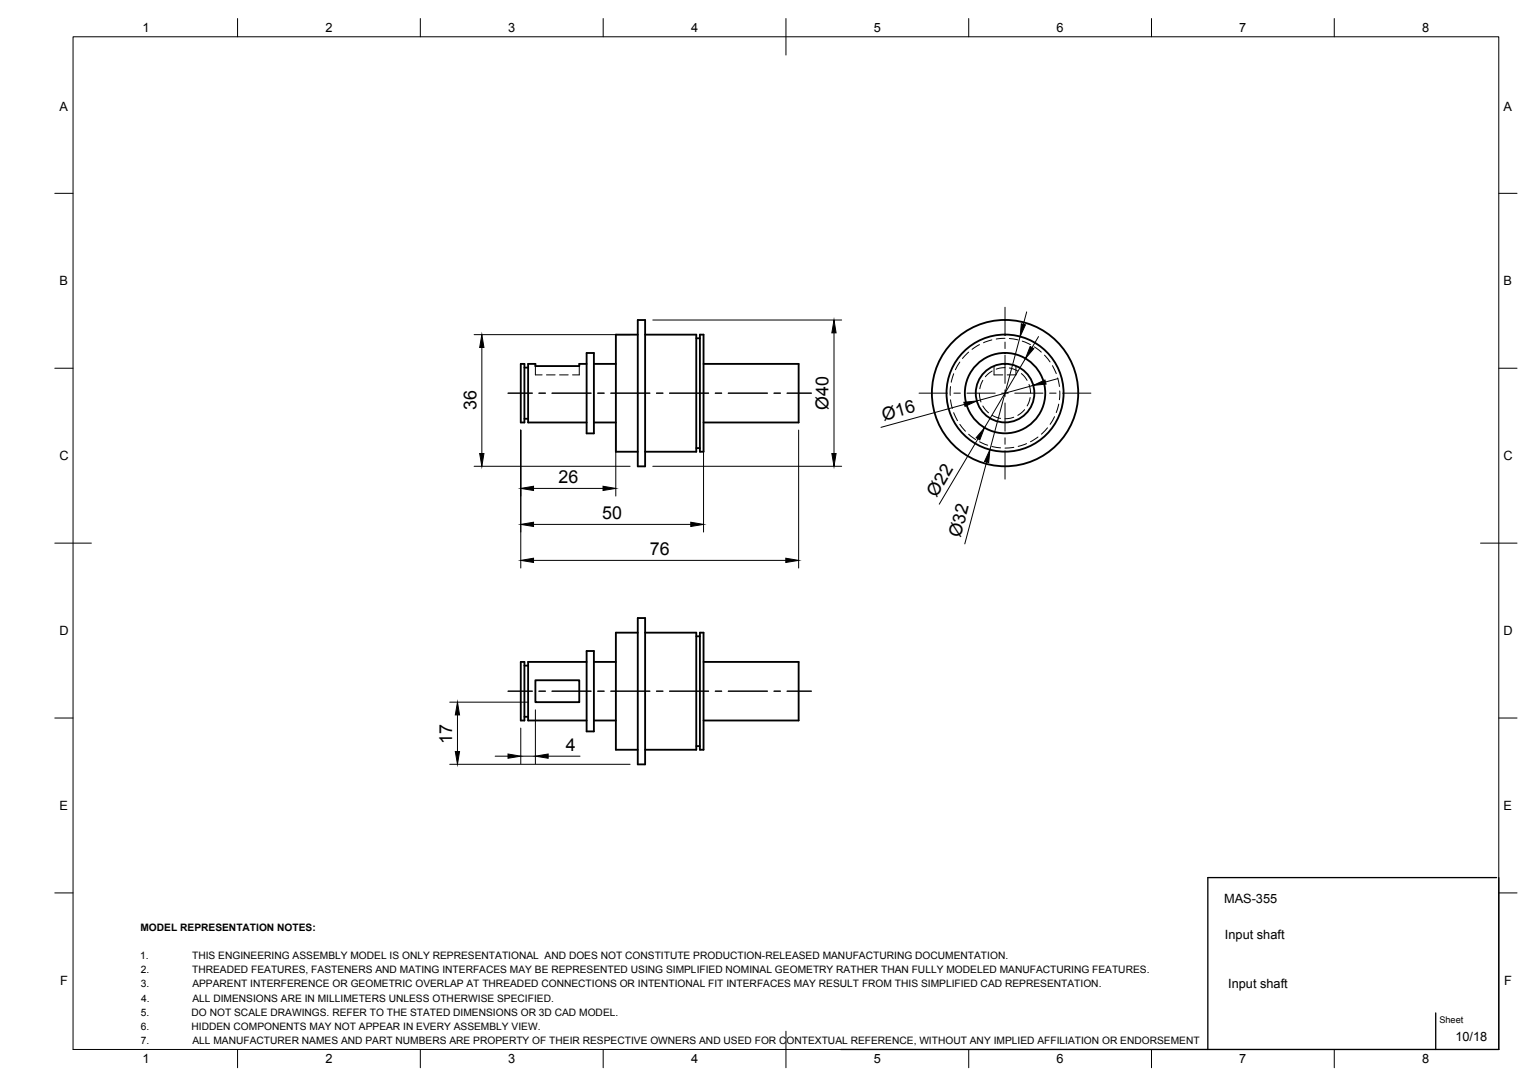
ISO-10303-21;
HEADER;
/* Generated by software containing ST-Developer
 * from STEP Tools, Inc. (www.steptools.com) 
 */

FILE_DESCRIPTION(
/* description */ ('Independent two-stage fixed-ring planetary gearbox,24/24/72 teeth,mod
ule2,20deg involutes,three planets per stage,4:1 x4:1=16:1. Native cut
-space/fillet/pattern tooth profiles derived from reusable gear blanks
; shared sun/planet/ring/carrier parts across both stages. Captured br
onze-journal input/carriers, headed retained planet pins, keyed inters
tage drive and modular keyed output interface. Native ideal gear links
; no torque, precision grade, production backlash/fits, lubrication, s
peed or life rating.'),
/* implementation_level */ '2;1');

FILE_NAME(
/* name */ 'Input shaft.step',
/* time_stamp */ '2026-11-08T19:10:00-08:00',
/* author */ (''),
/* organization */ (''),
/* preprocessor_version */ 'ST-DEVELOPER v20.2',
/* originating_system */ 'Autodesk Translation Framework v15.17.0.0',
/* authorisation */ '');

FILE_SCHEMA (('AUTOMOTIVE_DESIGN { 1 0 10303 214 3 1 1 }'));
ENDSEC;

DATA;
#10=MECHANICAL_DESIGN_GEOMETRIC_PRESENTATION_REPRESENTATION('',(#1166),#259224);
#1126=SHAPE_REPRESENTATION_RELATIONSHIP('SRR','None',#259373,#1146);
#1146=ADVANCED_BREP_SHAPE_REPRESENTATION('',(#1186),#259207);
#1166=STYLED_ITEM('',(#259482),#1186);
#1186=MANIFOLD_SOLID_BREP('Body1',#25153);
#1265=FACE_BOUND('',#3451,.T.);
#1266=FACE_BOUND('',#3453,.T.);
#1267=FACE_BOUND('',#3457,.T.);
#1268=FACE_BOUND('',#3459,.T.);
#1269=FACE_BOUND('',#3462,.T.);
#1270=FACE_BOUND('',#3464,.T.);
#1271=FACE_BOUND('',#3468,.T.);
#1272=FACE_BOUND('',#3470,.T.);
#1273=FACE_BOUND('',#3474,.T.);
#1274=FACE_BOUND('',#3480,.T.);
#1275=FACE_BOUND('',#3482,.T.);
#1509=PLANE('',#25812);
#1510=PLANE('',#25813);
#1511=PLANE('',#25815);
#1512=PLANE('',#25816);
#1513=PLANE('',#25817);
#1514=PLANE('',#25822);
#1515=PLANE('',#25824);
#1516=PLANE('',#25831);
#1517=PLANE('',#25833);
#1518=PLANE('',#25837);
#1519=PLANE('',#25840);
#1520=PLANE('',#25846);
#1521=PLANE('',#25849);
#1522=PLANE('',#25855);
#1523=PLANE('',#25859);
#1524=PLANE('',#25862);
#1525=PLANE('',#25863);
#2036=FACE_OUTER_BOUND('',#3444,.T.);
#2037=FACE_OUTER_BOUND('',#3445,.T.);
#2038=FACE_OUTER_BOUND('',#3446,.T.);
#2039=FACE_OUTER_BOUND('',#3447,.T.);
#2040=FACE_OUTER_BOUND('',#3448,.T.);
#2041=FACE_OUTER_BOUND('',#3449,.T.);
#2042=FACE_OUTER_BOUND('',#3450,.T.);
#2043=FACE_OUTER_BOUND('',#3452,.T.);
#2044=FACE_OUTER_BOUND('',#3454,.T.);
#2045=FACE_OUTER_BOUND('',#3455,.T.);
#2046=FACE_OUTER_BOUND('',#3456,.T.);
#2047=FACE_OUTER_BOUND('',#3458,.T.);
#2048=FACE_OUTER_BOUND('',#3460,.T.);
#2049=FACE_OUTER_BOUND('',#3461,.T.);
#2050=FACE_OUTER_BOUND('',#3463,.T.);
#2051=FACE_OUTER_BOUND('',#3465,.T.);
#2052=FACE_OUTER_BOUND('',#3466,.T.);
#2053=FACE_OUTER_BOUND('',#3467,.T.);
#2054=FACE_OUTER_BOUND('',#3469,.T.);
#2055=FACE_OUTER_BOUND('',#3471,.T.);
#2056=FACE_OUTER_BOUND('',#3472,.T.);
#2057=FACE_OUTER_BOUND('',#3473,.T.);
#2058=FACE_OUTER_BOUND('',#3475,.T.);
#2059=FACE_OUTER_BOUND('',#3476,.T.);
#2060=FACE_OUTER_BOUND('',#3477,.T.);
#2061=FACE_OUTER_BOUND('',#3478,.T.);
#2062=FACE_OUTER_BOUND('',#3479,.T.);
#2063=FACE_OUTER_BOUND('',#3481,.T.);
#3444=EDGE_LOOP('',(#17412,#17413,#17414,#17415));
#3445=EDGE_LOOP('',(#17416,#17417,#17418,#17419));
#3446=EDGE_LOOP('',(#17420,#17421,#17422,#17423));
#3447=EDGE_LOOP('',(#17424,#17425,#17426,#17427));
#3448=EDGE_LOOP('',(#17428,#17429,#17430,#17431));
#3449=EDGE_LOOP('',(#17432,#17433,#17434,#17435));
#3450=EDGE_LOOP('',(#17436));
#3451=EDGE_LOOP('',(#17437));
#3452=EDGE_LOOP('',(#17438));
#3453=EDGE_LOOP('',(#17439));
#3454=EDGE_LOOP('',(#17440,#17441,#17442,#17443));
#3455=EDGE_LOOP('',(#17444,#17445,#17446,#17447));
#3456=EDGE_LOOP('',(#17448));
#3457=EDGE_LOOP('',(#17449));
#3458=EDGE_LOOP('',(#17450));
#3459=EDGE_LOOP('',(#17451));
#3460=EDGE_LOOP('',(#17452,#17453,#17454,#17455));
#3461=EDGE_LOOP('',(#17456));
#3462=EDGE_LOOP('',(#17457));
#3463=EDGE_LOOP('',(#17458));
#3464=EDGE_LOOP('',(#17459));
#3465=EDGE_LOOP('',(#17460,#17461,#17462,#17463));
#3466=EDGE_LOOP('',(#17464,#17465,#17466,#17467));
#3467=EDGE_LOOP('',(#17468));
#3468=EDGE_LOOP('',(#17469));
#3469=EDGE_LOOP('',(#17470));
#3470=EDGE_LOOP('',(#17471));
#3471=EDGE_LOOP('',(#17472,#17473,#17474,#17475));
#3472=EDGE_LOOP('',(#17476,#17477,#17478,#17479));
#3473=EDGE_LOOP('',(#17480,#17481,#17482,#17483));
#3474=EDGE_LOOP('',(#17484,#17485,#17486,#17487));
#3475=EDGE_LOOP('',(#17488));
#3476=EDGE_LOOP('',(#17489,#17490,#17491,#17492));
#3477=EDGE_LOOP('',(#17493));
#3478=EDGE_LOOP('',(#17494,#17495,#17496,#17497));
#3479=EDGE_LOOP('',(#17498));
#3480=EDGE_LOOP('',(#17499));
#3481=EDGE_LOOP('',(#17500));
#3482=EDGE_LOOP('',(#17501));
#4599=CIRCLE('',#25814,8.);
#4600=CIRCLE('',#25818,8.);
#4601=CIRCLE('',#25820,7.);
#4602=CIRCLE('',#25821,7.);
#4603=CIRCLE('',#25823,8.);
#4604=CIRCLE('',#25825,8.);
#4605=CIRCLE('',#25827,8.);
#4606=CIRCLE('',#25829,15.);
#4607=CIRCLE('',#25830,15.);
#4608=CIRCLE('',#25832,16.);
#4609=CIRCLE('',#25834,16.);
#4610=CIRCLE('',#25836,16.);
#4611=CIRCLE('',#25838,11.);
#4612=CIRCLE('',#25839,8.);
#4613=CIRCLE('',#25841,11.);
#4614=CIRCLE('',#25842,8.);
#4615=CIRCLE('',#25845,8.);
#4616=CIRCLE('',#25847,20.);
#4617=CIRCLE('',#25848,16.);
#4618=CIRCLE('',#25850,20.);
#4619=CIRCLE('',#25853,16.);
#4620=CIRCLE('',#25857,8.);
#4621=CIRCLE('',#25858,8.);
#4622=CIRCLE('',#25861,16.);
#6959=LINE('',#52295,#8144);
#6960=LINE('',#52297,#8145);
#6961=LINE('',#52299,#8146);
#6962=LINE('',#52300,#8147);
#6963=LINE('',#52305,#8148);
#6964=LINE('',#52306,#8149);
#6965=LINE('',#52309,#8150);
#6966=LINE('',#52311,#8151);
#6967=LINE('',#52312,#8152);
#6968=LINE('',#52314,#8153);
#6969=LINE('',#52321,#8154);
#6970=LINE('',#52332,#8155);
#6971=LINE('',#52337,#8156);
#6972=LINE('',#52348,#8157);
#6973=LINE('',#52360,#8158);
#6974=LINE('',#52363,#8159);
#6975=LINE('',#52374,#8160);
#6976=LINE('',#52377,#8161);
#6977=LINE('',#52380,#8162);
#6978=LINE('',#52386,#8163);
#6979=LINE('',#52392,#8164);
#8144=VECTOR('',#28470,10.);
#8145=VECTOR('',#28471,10.);
#8146=VECTOR('',#28472,10.);
#8147=VECTOR('',#28473,10.);
#8148=VECTOR('',#28478,10.);
#8149=VECTOR('',#28479,10.);
#8150=VECTOR('',#28482,10.);
#8151=VECTOR('',#28483,10.);
#8152=VECTOR('',#28484,10.);
#8153=VECTOR('',#28487,10.);
#8154=VECTOR('',#28496,7.);
#8155=VECTOR('',#28511,8.);
#8156=VECTOR('',#28516,15.);
#8157=VECTOR('',#28531,16.);
#8158=VECTOR('',#28546,11.);
#8159=VECTOR('',#28549,8.);
#8160=VECTOR('',#28564,20.);
#8161=VECTOR('',#28567,16.);
#8162=VECTOR('',#28572,8.);
#8163=VECTOR('',#28579,8.);
#8164=VECTOR('',#28588,16.);
#9707=VERTEX_POINT('',#52293);
#9708=VERTEX_POINT('',#52294);
#9709=VERTEX_POINT('',#52296);
#9710=VERTEX_POINT('',#52298);
#9711=VERTEX_POINT('',#52302);
#9712=VERTEX_POINT('',#52304);
#9713=VERTEX_POINT('',#52308);
#9714=VERTEX_POINT('',#52310);
#9715=VERTEX_POINT('',#52318);
#9716=VERTEX_POINT('',#52320);
#9717=VERTEX_POINT('',#52324);
#9718=VERTEX_POINT('',#52327);
#9719=VERTEX_POINT('',#52330);
#9720=VERTEX_POINT('',#52334);
#9721=VERTEX_POINT('',#52336);
#9722=VERTEX_POINT('',#52340);
#9723=VERTEX_POINT('',#52343);
#9724=VERTEX_POINT('',#52346);
#9725=VERTEX_POINT('',#52350);
#9726=VERTEX_POINT('',#52352);
#9727=VERTEX_POINT('',#52355);
#9728=VERTEX_POINT('',#52357);
#9729=VERTEX_POINT('',#52362);
#9730=VERTEX_POINT('',#52366);
#9731=VERTEX_POINT('',#52368);
#9732=VERTEX_POINT('',#52371);
#9733=VERTEX_POINT('',#52376);
#9734=VERTEX_POINT('',#52383);
#9735=VERTEX_POINT('',#52385);
#9736=VERTEX_POINT('',#52390);
#12591=EDGE_CURVE('',#9707,#9708,#6959,.T.);
#12592=EDGE_CURVE('',#9707,#9709,#6960,.T.);
#12593=EDGE_CURVE('',#9710,#9709,#6961,.T.);
#12594=EDGE_CURVE('',#9710,#9708,#6962,.T.);
#12595=EDGE_CURVE('',#9708,#9711,#4599,.T.);
#12596=EDGE_CURVE('',#9712,#9710,#6963,.T.);
#12597=EDGE_CURVE('',#9711,#9712,#6964,.T.);
#12598=EDGE_CURVE('',#9711,#9713,#6965,.T.);
#12599=EDGE_CURVE('',#9712,#9714,#6966,.T.);
#12600=EDGE_CURVE('',#9714,#9713,#6967,.T.);
#12601=EDGE_CURVE('',#9709,#9714,#6968,.T.);
#12602=EDGE_CURVE('',#9713,#9707,#4600,.T.);
#12603=EDGE_CURVE('',#9715,#9715,#4601,.T.);
#12604=EDGE_CURVE('',#9715,#9716,#6969,.T.);
#12605=EDGE_CURVE('',#9716,#9716,#4602,.T.);
#12606=EDGE_CURVE('',#9717,#9717,#4603,.T.);
#12607=EDGE_CURVE('',#9718,#9718,#4604,.T.);
#12608=EDGE_CURVE('',#9719,#9719,#4605,.T.);
#12609=EDGE_CURVE('',#9719,#9718,#6970,.T.);
#12610=EDGE_CURVE('',#9720,#9720,#4606,.T.);
#12611=EDGE_CURVE('',#9720,#9721,#6971,.T.);
#12612=EDGE_CURVE('',#9721,#9721,#4607,.T.);
#12613=EDGE_CURVE('',#9722,#9722,#4608,.T.);
#12614=EDGE_CURVE('',#9723,#9723,#4609,.T.);
#12615=EDGE_CURVE('',#9724,#9724,#4610,.T.);
#12616=EDGE_CURVE('',#9724,#9723,#6972,.T.);
#12617=EDGE_CURVE('',#9725,#9725,#4611,.T.);
#12618=EDGE_CURVE('',#9726,#9726,#4612,.T.);
#12619=EDGE_CURVE('',#9727,#9727,#4613,.T.);
#12620=EDGE_CURVE('',#9728,#9728,#4614,.T.);
#12621=EDGE_CURVE('',#9725,#9727,#6973,.T.);
#12622=EDGE_CURVE('',#9728,#9729,#6974,.T.);
#12623=EDGE_CURVE('',#9729,#9729,#4615,.T.);
#12624=EDGE_CURVE('',#9730,#9730,#4616,.T.);
#12625=EDGE_CURVE('',#9731,#9731,#4617,.T.);
#12626=EDGE_CURVE('',#9732,#9732,#4618,.T.);
#12627=EDGE_CURVE('',#9730,#9732,#6975,.T.);
#12628=EDGE_CURVE('',#9722,#9733,#6976,.T.);
#12629=EDGE_CURVE('',#9733,#9733,#4619,.T.);
#12630=EDGE_CURVE('',#9717,#9726,#6977,.T.);
#12631=EDGE_CURVE('',#9734,#9734,#4620,.T.);
#12632=EDGE_CURVE('',#9734,#9735,#6978,.T.);
#12633=EDGE_CURVE('',#9735,#9735,#4621,.T.);
#12634=EDGE_CURVE('',#9736,#9736,#4622,.T.);
#12635=EDGE_CURVE('',#9736,#9731,#6979,.T.);
#17412=ORIENTED_EDGE('',*,*,#12591,.F.);
#17413=ORIENTED_EDGE('',*,*,#12592,.T.);
#17414=ORIENTED_EDGE('',*,*,#12593,.F.);
#17415=ORIENTED_EDGE('',*,*,#12594,.T.);
#17416=ORIENTED_EDGE('',*,*,#12595,.F.);
#17417=ORIENTED_EDGE('',*,*,#12594,.F.);
#17418=ORIENTED_EDGE('',*,*,#12596,.F.);
#17419=ORIENTED_EDGE('',*,*,#12597,.F.);
#17420=ORIENTED_EDGE('',*,*,#12598,.F.);
#17421=ORIENTED_EDGE('',*,*,#12597,.T.);
#17422=ORIENTED_EDGE('',*,*,#12599,.T.);
#17423=ORIENTED_EDGE('',*,*,#12600,.T.);
#17424=ORIENTED_EDGE('',*,*,#12596,.T.);
#17425=ORIENTED_EDGE('',*,*,#12593,.T.);
#17426=ORIENTED_EDGE('',*,*,#12601,.T.);
#17427=ORIENTED_EDGE('',*,*,#12599,.F.);
#17428=ORIENTED_EDGE('',*,*,#12602,.F.);
#17429=ORIENTED_EDGE('',*,*,#12600,.F.);
#17430=ORIENTED_EDGE('',*,*,#12601,.F.);
#17431=ORIENTED_EDGE('',*,*,#12592,.F.);
#17432=ORIENTED_EDGE('',*,*,#12603,.T.);
#17433=ORIENTED_EDGE('',*,*,#12604,.T.);
#17434=ORIENTED_EDGE('',*,*,#12605,.F.);
#17435=ORIENTED_EDGE('',*,*,#12604,.F.);
#17436=ORIENTED_EDGE('',*,*,#12606,.F.);
#17437=ORIENTED_EDGE('',*,*,#12603,.F.);
#17438=ORIENTED_EDGE('',*,*,#12607,.F.);
#17439=ORIENTED_EDGE('',*,*,#12605,.T.);
#17440=ORIENTED_EDGE('',*,*,#12608,.F.);
#17441=ORIENTED_EDGE('',*,*,#12609,.T.);
#17442=ORIENTED_EDGE('',*,*,#12607,.T.);
#17443=ORIENTED_EDGE('',*,*,#12609,.F.);
#17444=ORIENTED_EDGE('',*,*,#12610,.T.);
#17445=ORIENTED_EDGE('',*,*,#12611,.T.);
#17446=ORIENTED_EDGE('',*,*,#12612,.F.);
#17447=ORIENTED_EDGE('',*,*,#12611,.F.);
#17448=ORIENTED_EDGE('',*,*,#12613,.F.);
#17449=ORIENTED_EDGE('',*,*,#12610,.F.);
#17450=ORIENTED_EDGE('',*,*,#12614,.F.);
#17451=ORIENTED_EDGE('',*,*,#12612,.T.);
#17452=ORIENTED_EDGE('',*,*,#12615,.T.);
#17453=ORIENTED_EDGE('',*,*,#12616,.T.);
#17454=ORIENTED_EDGE('',*,*,#12614,.T.);
#17455=ORIENTED_EDGE('',*,*,#12616,.F.);
#17456=ORIENTED_EDGE('',*,*,#12617,.T.);
#17457=ORIENTED_EDGE('',*,*,#12618,.F.);
#17458=ORIENTED_EDGE('',*,*,#12619,.F.);
#17459=ORIENTED_EDGE('',*,*,#12620,.F.);
#17460=ORIENTED_EDGE('',*,*,#12617,.F.);
#17461=ORIENTED_EDGE('',*,*,#12621,.T.);
#17462=ORIENTED_EDGE('',*,*,#12619,.T.);
#17463=ORIENTED_EDGE('',*,*,#12621,.F.);
#17464=ORIENTED_EDGE('',*,*,#12620,.T.);
#17465=ORIENTED_EDGE('',*,*,#12622,.T.);
#17466=ORIENTED_EDGE('',*,*,#12623,.F.);
#17467=ORIENTED_EDGE('',*,*,#12622,.F.);
#17468=ORIENTED_EDGE('',*,*,#12624,.T.);
#17469=ORIENTED_EDGE('',*,*,#12625,.F.);
#17470=ORIENTED_EDGE('',*,*,#12626,.F.);
#17471=ORIENTED_EDGE('',*,*,#12615,.F.);
#17472=ORIENTED_EDGE('',*,*,#12624,.F.);
#17473=ORIENTED_EDGE('',*,*,#12627,.T.);
#17474=ORIENTED_EDGE('',*,*,#12626,.T.);
#17475=ORIENTED_EDGE('',*,*,#12627,.F.);
#17476=ORIENTED_EDGE('',*,*,#12613,.T.);
#17477=ORIENTED_EDGE('',*,*,#12628,.T.);
#17478=ORIENTED_EDGE('',*,*,#12629,.T.);
#17479=ORIENTED_EDGE('',*,*,#12628,.F.);
#17480=ORIENTED_EDGE('',*,*,#12606,.T.);
#17481=ORIENTED_EDGE('',*,*,#12630,.T.);
#17482=ORIENTED_EDGE('',*,*,#12618,.T.);
#17483=ORIENTED_EDGE('',*,*,#12630,.F.);
#17484=ORIENTED_EDGE('',*,*,#12598,.T.);
#17485=ORIENTED_EDGE('',*,*,#12602,.T.);
#17486=ORIENTED_EDGE('',*,*,#12591,.T.);
#17487=ORIENTED_EDGE('',*,*,#12595,.T.);
#17488=ORIENTED_EDGE('',*,*,#12608,.T.);
#17489=ORIENTED_EDGE('',*,*,#12631,.F.);
#17490=ORIENTED_EDGE('',*,*,#12632,.T.);
#17491=ORIENTED_EDGE('',*,*,#12633,.T.);
#17492=ORIENTED_EDGE('',*,*,#12632,.F.);
#17493=ORIENTED_EDGE('',*,*,#12633,.F.);
#17494=ORIENTED_EDGE('',*,*,#12634,.F.);
#17495=ORIENTED_EDGE('',*,*,#12635,.T.);
#17496=ORIENTED_EDGE('',*,*,#12625,.T.);
#17497=ORIENTED_EDGE('',*,*,#12635,.F.);
#17498=ORIENTED_EDGE('',*,*,#12634,.T.);
#17499=ORIENTED_EDGE('',*,*,#12623,.T.);
#17500=ORIENTED_EDGE('',*,*,#12629,.F.);
#17501=ORIENTED_EDGE('',*,*,#12631,.T.);
#23371=CYLINDRICAL_SURFACE('',#25819,7.);
#23372=CYLINDRICAL_SURFACE('',#25826,8.);
#23373=CYLINDRICAL_SURFACE('',#25828,15.);
#23374=CYLINDRICAL_SURFACE('',#25835,16.);
#23375=CYLINDRICAL_SURFACE('',#25843,11.);
#23376=CYLINDRICAL_SURFACE('',#25844,8.);
#23377=CYLINDRICAL_SURFACE('',#25851,20.);
#23378=CYLINDRICAL_SURFACE('',#25852,16.);
#23379=CYLINDRICAL_SURFACE('',#25854,8.);
#23380=CYLINDRICAL_SURFACE('',#25856,8.);
#23381=CYLINDRICAL_SURFACE('',#25860,16.);
#24142=ADVANCED_FACE('',(#2036),#1509,.F.);
#24143=ADVANCED_FACE('',(#2037),#1510,.F.);
#24144=ADVANCED_FACE('',(#2038),#1511,.F.);
#24145=ADVANCED_FACE('',(#2039),#1512,.F.);
#24146=ADVANCED_FACE('',(#2040),#1513,.F.);
#24147=ADVANCED_FACE('',(#2041),#23371,.T.);
#24148=ADVANCED_FACE('',(#2042,#1265),#1514,.F.);
#24149=ADVANCED_FACE('',(#2043,#1266),#1515,.F.);
#24150=ADVANCED_FACE('',(#2044),#23372,.T.);
#24151=ADVANCED_FACE('',(#2045),#23373,.T.);
#24152=ADVANCED_FACE('',(#2046,#1267),#1516,.F.);
#24153=ADVANCED_FACE('',(#2047,#1268),#1517,.F.);
#24154=ADVANCED_FACE('',(#2048),#23374,.T.);
#24155=ADVANCED_FACE('',(#2049,#1269),#1518,.T.);
#24156=ADVANCED_FACE('',(#2050,#1270),#1519,.F.);
#24157=ADVANCED_FACE('',(#2051),#23375,.T.);
#24158=ADVANCED_FACE('',(#2052),#23376,.T.);
#24159=ADVANCED_FACE('',(#2053,#1271),#1520,.T.);
#24160=ADVANCED_FACE('',(#2054,#1272),#1521,.F.);
#24161=ADVANCED_FACE('',(#2055),#23377,.T.);
#24162=ADVANCED_FACE('',(#2056),#23378,.T.);
#24163=ADVANCED_FACE('',(#2057,#1273),#23379,.T.);
#24164=ADVANCED_FACE('',(#2058),#1522,.T.);
#24165=ADVANCED_FACE('',(#2059),#23380,.T.);
#24166=ADVANCED_FACE('',(#2060),#1523,.F.);
#24167=ADVANCED_FACE('',(#2061),#23381,.T.);
#24168=ADVANCED_FACE('',(#2062,#1274),#1524,.T.);
#24169=ADVANCED_FACE('',(#2063,#1275),#1525,.F.);
#25153=CLOSED_SHELL('',(#24142,#24143,#24144,#24145,#24146,#24147,#24148,
#24149,#24150,#24151,#24152,#24153,#24154,#24155,#24156,#24157,#24158,#24159,
#24160,#24161,#24162,#24163,#24164,#24165,#24166,#24167,#24168,#24169));
#25811=AXIS2_PLACEMENT_3D('',#52291,#28466,#28467);
#25812=AXIS2_PLACEMENT_3D('',#52292,#28468,#28469);
#25813=AXIS2_PLACEMENT_3D('',#52301,#28474,#28475);
#25814=AXIS2_PLACEMENT_3D('',#52303,#28476,#28477);
#25815=AXIS2_PLACEMENT_3D('',#52307,#28480,#28481);
#25816=AXIS2_PLACEMENT_3D('',#52313,#28485,#28486);
#25817=AXIS2_PLACEMENT_3D('',#52315,#28488,#28489);
#25818=AXIS2_PLACEMENT_3D('',#52316,#28490,#28491);
#25819=AXIS2_PLACEMENT_3D('',#52317,#28492,#28493);
#25820=AXIS2_PLACEMENT_3D('',#52319,#28494,#28495);
#25821=AXIS2_PLACEMENT_3D('',#52322,#28497,#28498);
#25822=AXIS2_PLACEMENT_3D('',#52323,#28499,#28500);
#25823=AXIS2_PLACEMENT_3D('',#52325,#28501,#28502);
#25824=AXIS2_PLACEMENT_3D('',#52326,#28503,#28504);
#25825=AXIS2_PLACEMENT_3D('',#52328,#28505,#28506);
#25826=AXIS2_PLACEMENT_3D('',#52329,#28507,#28508);
#25827=AXIS2_PLACEMENT_3D('',#52331,#28509,#28510);
#25828=AXIS2_PLACEMENT_3D('',#52333,#28512,#28513);
#25829=AXIS2_PLACEMENT_3D('',#52335,#28514,#28515);
#25830=AXIS2_PLACEMENT_3D('',#52338,#28517,#28518);
#25831=AXIS2_PLACEMENT_3D('',#52339,#28519,#28520);
#25832=AXIS2_PLACEMENT_3D('',#52341,#28521,#28522);
#25833=AXIS2_PLACEMENT_3D('',#52342,#28523,#28524);
#25834=AXIS2_PLACEMENT_3D('',#52344,#28525,#28526);
#25835=AXIS2_PLACEMENT_3D('',#52345,#28527,#28528);
#25836=AXIS2_PLACEMENT_3D('',#52347,#28529,#28530);
#25837=AXIS2_PLACEMENT_3D('',#52349,#28532,#28533);
#25838=AXIS2_PLACEMENT_3D('',#52351,#28534,#28535);
#25839=AXIS2_PLACEMENT_3D('',#52353,#28536,#28537);
#25840=AXIS2_PLACEMENT_3D('',#52354,#28538,#28539);
#25841=AXIS2_PLACEMENT_3D('',#52356,#28540,#28541);
#25842=AXIS2_PLACEMENT_3D('',#52358,#28542,#28543);
#25843=AXIS2_PLACEMENT_3D('',#52359,#28544,#28545);
#25844=AXIS2_PLACEMENT_3D('',#52361,#28547,#28548);
#25845=AXIS2_PLACEMENT_3D('',#52364,#28550,#28551);
#25846=AXIS2_PLACEMENT_3D('',#52365,#28552,#28553);
#25847=AXIS2_PLACEMENT_3D('',#52367,#28554,#28555);
#25848=AXIS2_PLACEMENT_3D('',#52369,#28556,#28557);
#25849=AXIS2_PLACEMENT_3D('',#52370,#28558,#28559);
#25850=AXIS2_PLACEMENT_3D('',#52372,#28560,#28561);
#25851=AXIS2_PLACEMENT_3D('',#52373,#28562,#28563);
#25852=AXIS2_PLACEMENT_3D('',#52375,#28565,#28566);
#25853=AXIS2_PLACEMENT_3D('',#52378,#28568,#28569);
#25854=AXIS2_PLACEMENT_3D('',#52379,#28570,#28571);
#25855=AXIS2_PLACEMENT_3D('',#52381,#28573,#28574);
#25856=AXIS2_PLACEMENT_3D('',#52382,#28575,#28576);
#25857=AXIS2_PLACEMENT_3D('',#52384,#28577,#28578);
#25858=AXIS2_PLACEMENT_3D('',#52387,#28580,#28581);
#25859=AXIS2_PLACEMENT_3D('',#52388,#28582,#28583);
#25860=AXIS2_PLACEMENT_3D('',#52389,#28584,#28585);
#25861=AXIS2_PLACEMENT_3D('',#52391,#28586,#28587);
#25862=AXIS2_PLACEMENT_3D('',#52393,#28589,#28590);
#25863=AXIS2_PLACEMENT_3D('',#52394,#28591,#28592);
#28466=DIRECTION('axis',(0.,0.,1.));
#28467=DIRECTION('refdir',(1.,0.,0.));
#28468=DIRECTION('center_axis',(0.,-1.,0.));
#28469=DIRECTION('ref_axis',(-1.,0.,0.));
#28470=DIRECTION('',(0.,0.,1.));
#28471=DIRECTION('',(-1.,0.,0.));
#28472=DIRECTION('',(0.,0.,-1.));
#28473=DIRECTION('',(1.,0.,0.));
#28474=DIRECTION('center_axis',(0.,0.,1.));
#28475=DIRECTION('ref_axis',(1.,0.,0.));
#28476=DIRECTION('center_axis',(0.,0.,1.));
#28477=DIRECTION('ref_axis',(1.,0.,0.));
#28478=DIRECTION('',(0.,-1.,0.));
#28479=DIRECTION('',(-1.,0.,0.));
#28480=DIRECTION('center_axis',(0.,1.,0.));
#28481=DIRECTION('ref_axis',(1.,0.,0.));
#28482=DIRECTION('',(0.,0.,-1.));
#28483=DIRECTION('',(0.,0.,-1.));
#28484=DIRECTION('',(1.,0.,0.));
#28485=DIRECTION('center_axis',(-1.,0.,0.));
#28486=DIRECTION('ref_axis',(0.,1.,0.));
#28487=DIRECTION('',(0.,1.,0.));
#28488=DIRECTION('center_axis',(0.,0.,-1.));
#28489=DIRECTION('ref_axis',(-1.,0.,0.));
#28490=DIRECTION('center_axis',(0.,0.,-1.));
#28491=DIRECTION('ref_axis',(1.,0.,0.));
#28492=DIRECTION('center_axis',(0.,0.,1.));
#28493=DIRECTION('ref_axis',(1.,0.,0.));
#28494=DIRECTION('center_axis',(0.,0.,1.));
#28495=DIRECTION('ref_axis',(1.,0.,0.));
#28496=DIRECTION('',(0.,0.,1.));
#28497=DIRECTION('center_axis',(0.,0.,1.));
#28498=DIRECTION('ref_axis',(1.,0.,0.));
#28499=DIRECTION('center_axis',(0.,0.,-1.));
#28500=DIRECTION('ref_axis',(-1.,0.,0.));
#28501=DIRECTION('center_axis',(0.,0.,-1.));
#28502=DIRECTION('ref_axis',(1.,0.,0.));
#28503=DIRECTION('center_axis',(0.,0.,1.));
#28504=DIRECTION('ref_axis',(1.,0.,0.));
#28505=DIRECTION('center_axis',(0.,0.,1.));
#28506=DIRECTION('ref_axis',(1.,0.,0.));
#28507=DIRECTION('center_axis',(0.,0.,1.));
#28508=DIRECTION('ref_axis',(1.,0.,0.));
#28509=DIRECTION('center_axis',(0.,0.,1.));
#28510=DIRECTION('ref_axis',(1.,0.,0.));
#28511=DIRECTION('',(0.,0.,-1.));
#28512=DIRECTION('center_axis',(0.,0.,1.));
#28513=DIRECTION('ref_axis',(1.,0.,0.));
#28514=DIRECTION('center_axis',(0.,0.,1.));
#28515=DIRECTION('ref_axis',(1.,0.,0.));
#28516=DIRECTION('',(0.,0.,1.));
#28517=DIRECTION('center_axis',(0.,0.,1.));
#28518=DIRECTION('ref_axis',(1.,0.,0.));
#28519=DIRECTION('center_axis',(0.,0.,-1.));
#28520=DIRECTION('ref_axis',(-1.,0.,0.));
#28521=DIRECTION('center_axis',(0.,0.,-1.));
#28522=DIRECTION('ref_axis',(1.,0.,0.));
#28523=DIRECTION('center_axis',(0.,0.,1.));
#28524=DIRECTION('ref_axis',(1.,0.,0.));
#28525=DIRECTION('center_axis',(0.,0.,1.));
#28526=DIRECTION('ref_axis',(1.,0.,0.));
#28527=DIRECTION('center_axis',(0.,0.,1.));
#28528=DIRECTION('ref_axis',(1.,0.,0.));
#28529=DIRECTION('center_axis',(0.,0.,-1.));
#28530=DIRECTION('ref_axis',(1.,0.,0.));
#28531=DIRECTION('',(0.,0.,-1.));
#28532=DIRECTION('center_axis',(0.,0.,1.));
#28533=DIRECTION('ref_axis',(1.,0.,0.));
#28534=DIRECTION('center_axis',(0.,0.,1.));
#28535=DIRECTION('ref_axis',(1.,0.,0.));
#28536=DIRECTION('center_axis',(0.,0.,1.));
#28537=DIRECTION('ref_axis',(1.,0.,0.));
#28538=DIRECTION('center_axis',(0.,0.,1.));
#28539=DIRECTION('ref_axis',(1.,0.,0.));
#28540=DIRECTION('center_axis',(0.,0.,1.));
#28541=DIRECTION('ref_axis',(1.,0.,0.));
#28542=DIRECTION('center_axis',(0.,0.,-1.));
#28543=DIRECTION('ref_axis',(1.,0.,0.));
#28544=DIRECTION('center_axis',(0.,0.,1.));
#28545=DIRECTION('ref_axis',(1.,0.,0.));
#28546=DIRECTION('',(0.,0.,-1.));
#28547=DIRECTION('center_axis',(0.,0.,1.));
#28548=DIRECTION('ref_axis',(1.,0.,0.));
#28549=DIRECTION('',(0.,0.,-1.));
#28550=DIRECTION('center_axis',(0.,0.,-1.));
#28551=DIRECTION('ref_axis',(1.,0.,0.));
#28552=DIRECTION('center_axis',(0.,0.,1.));
#28553=DIRECTION('ref_axis',(1.,0.,0.));
#28554=DIRECTION('center_axis',(0.,0.,1.));
#28555=DIRECTION('ref_axis',(1.,0.,0.));
#28556=DIRECTION('center_axis',(0.,0.,1.));
#28557=DIRECTION('ref_axis',(1.,0.,0.));
#28558=DIRECTION('center_axis',(0.,0.,1.));
#28559=DIRECTION('ref_axis',(1.,0.,0.));
#28560=DIRECTION('center_axis',(0.,0.,1.));
#28561=DIRECTION('ref_axis',(1.,0.,0.));
#28562=DIRECTION('center_axis',(0.,0.,1.));
#28563=DIRECTION('ref_axis',(1.,0.,0.));
#28564=DIRECTION('',(0.,0.,-1.));
#28565=DIRECTION('center_axis',(0.,0.,1.));
#28566=DIRECTION('ref_axis',(1.,0.,0.));
#28567=DIRECTION('',(0.,0.,-1.));
#28568=DIRECTION('center_axis',(0.,0.,1.));
#28569=DIRECTION('ref_axis',(1.,0.,0.));
#28570=DIRECTION('center_axis',(0.,0.,1.));
#28571=DIRECTION('ref_axis',(1.,0.,0.));
#28572=DIRECTION('',(0.,0.,-1.));
#28573=DIRECTION('center_axis',(0.,0.,1.));
#28574=DIRECTION('ref_axis',(1.,0.,0.));
#28575=DIRECTION('center_axis',(0.,0.,1.));
#28576=DIRECTION('ref_axis',(1.,0.,0.));
#28577=DIRECTION('center_axis',(0.,0.,1.));
#28578=DIRECTION('ref_axis',(1.,0.,0.));
#28579=DIRECTION('',(0.,0.,-1.));
#28580=DIRECTION('center_axis',(0.,0.,1.));
#28581=DIRECTION('ref_axis',(1.,0.,0.));
#28582=DIRECTION('center_axis',(0.,0.,1.));
#28583=DIRECTION('ref_axis',(1.,0.,0.));
#28584=DIRECTION('center_axis',(0.,0.,1.));
#28585=DIRECTION('ref_axis',(1.,0.,0.));
#28586=DIRECTION('center_axis',(0.,0.,1.));
#28587=DIRECTION('ref_axis',(1.,0.,0.));
#28588=DIRECTION('',(0.,0.,-1.));
#28589=DIRECTION('center_axis',(0.,0.,1.));
#28590=DIRECTION('ref_axis',(1.,0.,0.));
#28591=DIRECTION('center_axis',(0.,0.,1.));
#28592=DIRECTION('ref_axis',(1.,0.,0.));
#52291=CARTESIAN_POINT('',(0.,0.,0.));
#52292=CARTESIAN_POINT('Origin',(11.,-3.,42.));
#52293=CARTESIAN_POINT('',(7.41619848709566,-3.,30.));
#52294=CARTESIAN_POINT('',(7.41619848709566,-3.,42.));
#52295=CARTESIAN_POINT('',(7.41619848709566,-3.,20.));
#52296=CARTESIAN_POINT('',(5.,-3.,30.));
#52297=CARTESIAN_POINT('',(5.,-3.,30.));
#52298=CARTESIAN_POINT('',(5.,-3.,42.));
#52299=CARTESIAN_POINT('',(5.,-3.,42.));
#52300=CARTESIAN_POINT('',(5.,-3.,42.));
#52301=CARTESIAN_POINT('Origin',(8.,0.,42.));
#52302=CARTESIAN_POINT('',(7.41619848709566,3.,42.));
#52303=CARTESIAN_POINT('Origin',(0.,0.,42.));
#52304=CARTESIAN_POINT('',(5.,3.,42.));
#52305=CARTESIAN_POINT('',(5.,3.,42.));
#52306=CARTESIAN_POINT('',(11.,3.,42.));
#52307=CARTESIAN_POINT('Origin',(5.,3.,42.));
#52308=CARTESIAN_POINT('',(7.41619848709566,3.,30.));
#52309=CARTESIAN_POINT('',(7.41619848709566,3.,20.));
#52310=CARTESIAN_POINT('',(5.,3.,30.));
#52311=CARTESIAN_POINT('',(5.,3.,42.));
#52312=CARTESIAN_POINT('',(11.,3.,30.));
#52313=CARTESIAN_POINT('Origin',(5.,-3.,42.));
#52314=CARTESIAN_POINT('',(5.,3.,30.));
#52315=CARTESIAN_POINT('Origin',(8.,0.,30.));
#52316=CARTESIAN_POINT('Origin',(0.,0.,30.));
#52317=CARTESIAN_POINT('Origin',(0.,0.,44.5));
#52318=CARTESIAN_POINT('',(-7.,-8.57252759403147E-16,44.));
#52319=CARTESIAN_POINT('Origin',(0.,0.,44.));
#52320=CARTESIAN_POINT('',(-7.,-8.57252759403147E-16,45.));
#52321=CARTESIAN_POINT('',(-7.,-8.57252759403147E-16,44.5));
#52322=CARTESIAN_POINT('Origin',(0.,0.,45.));
#52323=CARTESIAN_POINT('Origin',(11.,0.,44.));
#52324=CARTESIAN_POINT('',(-8.,9.79717439317883E-16,44.));
#52325=CARTESIAN_POINT('Origin',(0.,0.,44.));
#52326=CARTESIAN_POINT('Origin',(7.,0.,45.));
#52327=CARTESIAN_POINT('',(-8.,-9.79717439317883E-16,45.));
#52328=CARTESIAN_POINT('Origin',(0.,0.,45.));
#52329=CARTESIAN_POINT('Origin',(0.,0.,20.));
#52330=CARTESIAN_POINT('',(-8.,-9.79717439317883E-16,46.));
#52331=CARTESIAN_POINT('Origin',(0.,0.,46.));
#52332=CARTESIAN_POINT('',(-8.,-9.79717439317883E-16,20.));
#52333=CARTESIAN_POINT('Origin',(0.,0.,-2.5));
#52334=CARTESIAN_POINT('',(-15.,-1.83697019872103E-15,-3.));
#52335=CARTESIAN_POINT('Origin',(0.,0.,-3.));
#52336=CARTESIAN_POINT('',(-15.,-1.83697019872103E-15,-2.));
#52337=CARTESIAN_POINT('',(-15.,-1.83697019872103E-15,-2.5));
#52338=CARTESIAN_POINT('Origin',(0.,0.,-2.));
#52339=CARTESIAN_POINT('Origin',(19.,0.,-3.));
#52340=CARTESIAN_POINT('',(-16.,1.95943487863577E-15,-3.));
#52341=CARTESIAN_POINT('Origin',(0.,0.,-3.));
#52342=CARTESIAN_POINT('Origin',(15.,0.,-2.));
#52343=CARTESIAN_POINT('',(-16.,-1.95943487863577E-15,-2.));
#52344=CARTESIAN_POINT('Origin',(0.,0.,-2.));
#52345=CARTESIAN_POINT('Origin',(0.,0.,-4.));
#52346=CARTESIAN_POINT('',(-16.,1.95943487863577E-15,12.));
#52347=CARTESIAN_POINT('Origin',(0.,0.,12.));
#52348=CARTESIAN_POINT('',(-16.,-1.95943487863577E-15,-4.));
#52349=CARTESIAN_POINT('Origin',(0.,0.,28.));
#52350=CARTESIAN_POINT('',(-11.,-1.34711147906209E-15,28.));
#52351=CARTESIAN_POINT('Origin',(0.,0.,28.));
#52352=CARTESIAN_POINT('',(-8.,-9.79717439317883E-16,28.));
#52353=CARTESIAN_POINT('Origin',(0.,0.,28.));
#52354=CARTESIAN_POINT('Origin',(0.,0.,26.));
#52355=CARTESIAN_POINT('',(-11.,-1.34711147906209E-15,26.));
#52356=CARTESIAN_POINT('Origin',(0.,0.,26.));
#52357=CARTESIAN_POINT('',(-8.,9.79717439317883E-16,26.));
#52358=CARTESIAN_POINT('Origin',(0.,0.,26.));
#52359=CARTESIAN_POINT('Origin',(0.,0.,26.));
#52360=CARTESIAN_POINT('',(-11.,-1.34711147906209E-15,26.));
#52361=CARTESIAN_POINT('Origin',(0.,0.,20.));
#52362=CARTESIAN_POINT('',(-8.,-9.79717439317883E-16,20.));
#52363=CARTESIAN_POINT('',(-8.,-9.79717439317883E-16,20.));
#52364=CARTESIAN_POINT('Origin',(0.,0.,20.));
#52365=CARTESIAN_POINT('Origin',(0.,0.,14.));
#52366=CARTESIAN_POINT('',(-20.,-2.44929359829471E-15,14.));
#52367=CARTESIAN_POINT('Origin',(0.,0.,14.));
#52368=CARTESIAN_POINT('',(-16.,-1.95943487863577E-15,14.));
#52369=CARTESIAN_POINT('Origin',(0.,0.,14.));
#52370=CARTESIAN_POINT('Origin',(0.,0.,12.));
#52371=CARTESIAN_POINT('',(-20.,-2.44929359829471E-15,12.));
#52372=CARTESIAN_POINT('Origin',(0.,0.,12.));
#52373=CARTESIAN_POINT('Origin',(0.,0.,12.));
#52374=CARTESIAN_POINT('',(-20.,-2.44929359829471E-15,12.));
#52375=CARTESIAN_POINT('Origin',(0.,0.,-4.));
#52376=CARTESIAN_POINT('',(-16.,-1.95943487863577E-15,-4.));
#52377=CARTESIAN_POINT('',(-16.,-1.95943487863577E-15,-4.));
#52378=CARTESIAN_POINT('Origin',(0.,0.,-4.));
#52379=CARTESIAN_POINT('Origin',(0.,0.,20.));
#52380=CARTESIAN_POINT('',(-8.,-9.79717439317883E-16,20.));
#52381=CARTESIAN_POINT('Origin',(0.,0.,46.));
#52382=CARTESIAN_POINT('Origin',(0.,0.,-20.));
#52383=CARTESIAN_POINT('',(-8.,-9.79717439317883E-16,-4.));
#52384=CARTESIAN_POINT('Origin',(0.,0.,-4.));
#52385=CARTESIAN_POINT('',(-8.,-9.79717439317883E-16,-30.));
#52386=CARTESIAN_POINT('',(-8.,-9.79717439317883E-16,-20.));
#52387=CARTESIAN_POINT('Origin',(0.,0.,-30.));
#52388=CARTESIAN_POINT('Origin',(0.,0.,-30.));
#52389=CARTESIAN_POINT('Origin',(0.,0.,-4.));
#52390=CARTESIAN_POINT('',(-16.,-1.95943487863577E-15,20.));
#52391=CARTESIAN_POINT('Origin',(0.,0.,20.));
#52392=CARTESIAN_POINT('',(-16.,-1.95943487863577E-15,-4.));
#52393=CARTESIAN_POINT('Origin',(0.,0.,20.));
#52394=CARTESIAN_POINT('Origin',(0.,0.,-4.));
#259185=UNCERTAINTY_MEASURE_WITH_UNIT(LENGTH_MEASURE(0.01),#259225,
'DISTANCE_ACCURACY_VALUE',
'Maximum model space distance between geometric entities at asserted c
onnectivities');
#259202=UNCERTAINTY_MEASURE_WITH_UNIT(LENGTH_MEASURE(0.01),#259225,
'DISTANCE_ACCURACY_VALUE',
'Maximum model space distance between geometric entities at asserted c
onnectivities');
#259207=(
GEOMETRIC_REPRESENTATION_CONTEXT(3)
GLOBAL_UNCERTAINTY_ASSIGNED_CONTEXT((#259185))
GLOBAL_UNIT_ASSIGNED_CONTEXT((#259225,#259227,#259228))
REPRESENTATION_CONTEXT('','3D')
);
#259224=(
GEOMETRIC_REPRESENTATION_CONTEXT(3)
GLOBAL_UNCERTAINTY_ASSIGNED_CONTEXT((#259202))
GLOBAL_UNIT_ASSIGNED_CONTEXT((#259225,#259227,#259228))
REPRESENTATION_CONTEXT('','3D')
);
#259225=(
LENGTH_UNIT()
NAMED_UNIT(*)
SI_UNIT(.MILLI.,.METRE.)
);
#259227=(
NAMED_UNIT(*)
PLANE_ANGLE_UNIT()
SI_UNIT($,.RADIAN.)
);
#259228=(
NAMED_UNIT(*)
SI_UNIT($,.STERADIAN.)
SOLID_ANGLE_UNIT()
);
#259233=SHAPE_DEFINITION_REPRESENTATION(#259254,#259373);
#259254=PRODUCT_DEFINITION_SHAPE('',$,#259395);
#259373=SHAPE_REPRESENTATION('',(#25811),#259207);
#259390=PRODUCT_DEFINITION_CONTEXT('part definition',#259455,'design');
#259395=PRODUCT_DEFINITION('Input shaft','Input shaft',#259416,#259390);
#259416=PRODUCT_DEFINITION_FORMATION('',$,#259461);
#259455=APPLICATION_CONTEXT(
'Core Data for Automotive Mechanical Design Process');
#259456=PRODUCT_CONTEXT('part definition',#259455,'mechanical');
#259461=PRODUCT('Input shaft','Input shaft','Input shaft',(#259456));
#259482=PRESENTATION_STYLE_ASSIGNMENT((#259497));
#259497=SURFACE_STYLE_USAGE(.BOTH.,#259512);
#259512=SURFACE_SIDE_STYLE('',(#259527));
#259527=SURFACE_STYLE_FILL_AREA(#259542);
#259542=FILL_AREA_STYLE('Shaft gray',(#259557));
#259557=FILL_AREA_STYLE_COLOUR('Shaft gray',#259572);
#259572=COLOUR_RGB('Shaft gray',0.576470588235294,0.615686274509804,0.666666666666667);
ENDSEC;
END-ISO-10303-21;
